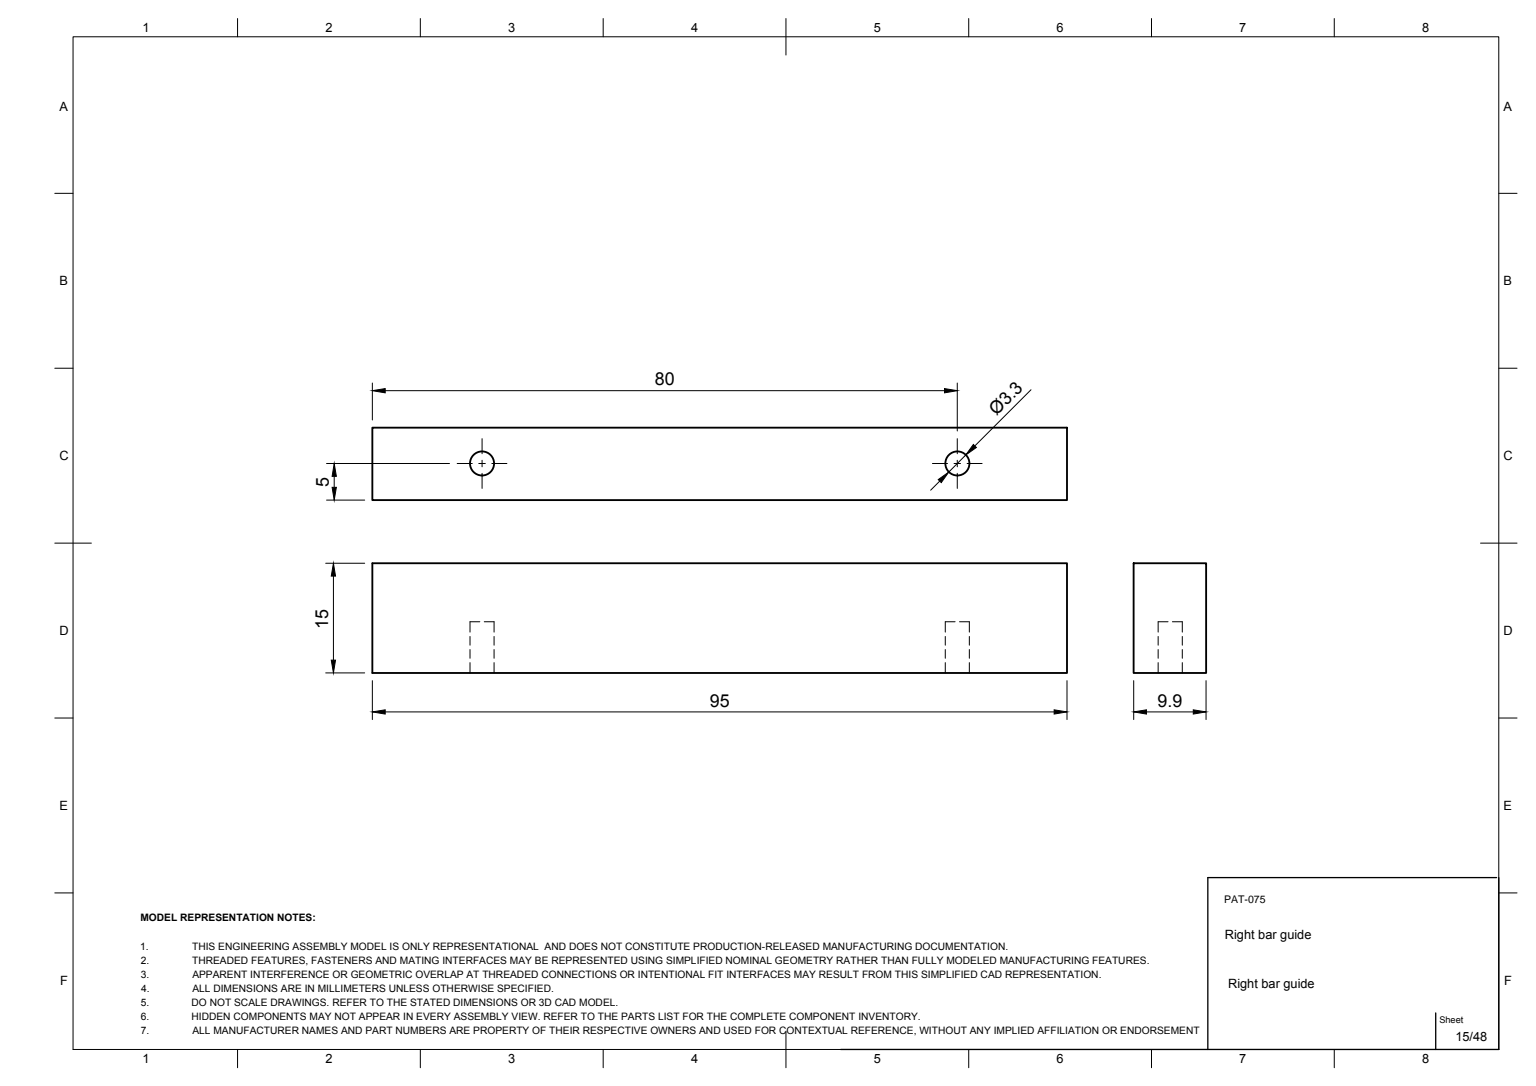
ISO-10303-21;
HEADER;
/* Generated by software containing ST-Developer
 * from STEP Tools, Inc. (www.steptools.com) 
 */

FILE_DESCRIPTION(
/* description */ ('Over-Centre Plunger Toggle Clamp on Slotted Fixture Frame'),
/* implementation_level */ '2;1');

FILE_NAME(
/* name */ 
'Right bar guide.step',
/* time_stamp */ '2026-10-28T03:23:24-07:00',
/* author */ (''),
/* organization */ (''),
/* preprocessor_version */ 'ST-DEVELOPER v20.2',
/* originating_system */ 'Autodesk Translation Framework v15.17.0.0',
/* authorisation */ '');

FILE_SCHEMA (('AUTOMOTIVE_DESIGN { 1 0 10303 214 3 1 1 }'));
ENDSEC;

DATA;
#10=MECHANICAL_DESIGN_GEOMETRIC_PRESENTATION_REPRESENTATION('',(#523),#15212);
#439=SHAPE_REPRESENTATION_RELATIONSHIP('SRR','None',#15413,#481);
#481=ADVANCED_BREP_SHAPE_REPRESENTATION('',(#574),#15175);
#523=STYLED_ITEM('',(#15733),#574);
#574=MANIFOLD_SOLID_BREP('Body1',#8255);
#710=FACE_BOUND('',#1814,.T.);
#711=FACE_BOUND('',#1815,.T.);
#854=PLANE('',#9033);
#855=PLANE('',#9037);
#856=PLANE('',#9038);
#857=PLANE('',#9039);
#858=PLANE('',#9040);
#859=PLANE('',#9041);
#860=PLANE('',#9042);
#861=PLANE('',#9043);
#1219=FACE_OUTER_BOUND('',#1804,.T.);
#1220=FACE_OUTER_BOUND('',#1805,.T.);
#1221=FACE_OUTER_BOUND('',#1806,.T.);
#1222=FACE_OUTER_BOUND('',#1807,.T.);
#1223=FACE_OUTER_BOUND('',#1808,.T.);
#1224=FACE_OUTER_BOUND('',#1809,.T.);
#1225=FACE_OUTER_BOUND('',#1810,.T.);
#1226=FACE_OUTER_BOUND('',#1811,.T.);
#1227=FACE_OUTER_BOUND('',#1812,.T.);
#1228=FACE_OUTER_BOUND('',#1813,.T.);
#1804=EDGE_LOOP('',(#6151,#6152,#6153,#6154));
#1805=EDGE_LOOP('',(#6155));
#1806=EDGE_LOOP('',(#6156,#6157,#6158,#6159));
#1807=EDGE_LOOP('',(#6160));
#1808=EDGE_LOOP('',(#6161,#6162,#6163,#6164));
#1809=EDGE_LOOP('',(#6165,#6166,#6167,#6168));
#1810=EDGE_LOOP('',(#6169,#6170,#6171,#6172));
#1811=EDGE_LOOP('',(#6173,#6174,#6175,#6176));
#1812=EDGE_LOOP('',(#6177,#6178,#6179,#6180));
#1813=EDGE_LOOP('',(#6181,#6182,#6183,#6184));
#1814=EDGE_LOOP('',(#6185));
#1815=EDGE_LOOP('',(#6186));
#2400=LINE('',#13000,#3030);
#2401=LINE('',#13007,#3031);
#2402=LINE('',#13013,#3032);
#2403=LINE('',#13015,#3033);
#2404=LINE('',#13017,#3034);
#2405=LINE('',#13018,#3035);
#2406=LINE('',#13021,#3036);
#2407=LINE('',#13023,#3037);
#2408=LINE('',#13024,#3038);
#2409=LINE('',#13027,#3039);
#2410=LINE('',#13029,#3040);
#2411=LINE('',#13030,#3041);
#2412=LINE('',#13032,#3042);
#2413=LINE('',#13033,#3043);
#3030=VECTOR('',#10461,0.165);
#3031=VECTOR('',#10470,0.165);
#3032=VECTOR('',#10477,1.);
#3033=VECTOR('',#10478,1.);
#3034=VECTOR('',#10479,1.);
#3035=VECTOR('',#10480,1.);
#3036=VECTOR('',#10483,1.);
#3037=VECTOR('',#10484,1.);
#3038=VECTOR('',#10485,1.);
#3039=VECTOR('',#10488,1.);
#3040=VECTOR('',#10489,1.);
#3041=VECTOR('',#10490,1.);
#3042=VECTOR('',#10493,1.);
#3043=VECTOR('',#10494,1.);
#3613=CIRCLE('',#9031,0.165);
#3614=CIRCLE('',#9032,0.165);
#3615=CIRCLE('',#9035,0.165);
#3616=CIRCLE('',#9036,0.165);
#4053=VERTEX_POINT('',#12997);
#4054=VERTEX_POINT('',#12999);
#4055=VERTEX_POINT('',#13004);
#4056=VERTEX_POINT('',#13006);
#4057=VERTEX_POINT('',#13011);
#4058=VERTEX_POINT('',#13012);
#4059=VERTEX_POINT('',#13014);
#4060=VERTEX_POINT('',#13016);
#4061=VERTEX_POINT('',#13020);
#4062=VERTEX_POINT('',#13022);
#4063=VERTEX_POINT('',#13026);
#4064=VERTEX_POINT('',#13028);
#4836=EDGE_CURVE('',#4053,#4053,#3613,.T.);
#4837=EDGE_CURVE('',#4053,#4054,#2400,.T.);
#4838=EDGE_CURVE('',#4054,#4054,#3614,.T.);
#4839=EDGE_CURVE('',#4055,#4055,#3615,.T.);
#4840=EDGE_CURVE('',#4055,#4056,#2401,.T.);
#4841=EDGE_CURVE('',#4056,#4056,#3616,.T.);
#4842=EDGE_CURVE('',#4057,#4058,#2402,.T.);
#4843=EDGE_CURVE('',#4058,#4059,#2403,.T.);
#4844=EDGE_CURVE('',#4060,#4059,#2404,.T.);
#4845=EDGE_CURVE('',#4057,#4060,#2405,.T.);
#4846=EDGE_CURVE('',#4061,#4057,#2406,.T.);
#4847=EDGE_CURVE('',#4062,#4060,#2407,.T.);
#4848=EDGE_CURVE('',#4061,#4062,#2408,.T.);
#4849=EDGE_CURVE('',#4063,#4061,#2409,.T.);
#4850=EDGE_CURVE('',#4064,#4062,#2410,.T.);
#4851=EDGE_CURVE('',#4063,#4064,#2411,.T.);
#4852=EDGE_CURVE('',#4058,#4063,#2412,.T.);
#4853=EDGE_CURVE('',#4059,#4064,#2413,.T.);
#6151=ORIENTED_EDGE('',*,*,#4836,.F.);
#6152=ORIENTED_EDGE('',*,*,#4837,.T.);
#6153=ORIENTED_EDGE('',*,*,#4838,.T.);
#6154=ORIENTED_EDGE('',*,*,#4837,.F.);
#6155=ORIENTED_EDGE('',*,*,#4838,.F.);
#6156=ORIENTED_EDGE('',*,*,#4839,.F.);
#6157=ORIENTED_EDGE('',*,*,#4840,.T.);
#6158=ORIENTED_EDGE('',*,*,#4841,.T.);
#6159=ORIENTED_EDGE('',*,*,#4840,.F.);
#6160=ORIENTED_EDGE('',*,*,#4841,.F.);
#6161=ORIENTED_EDGE('',*,*,#4842,.T.);
#6162=ORIENTED_EDGE('',*,*,#4843,.T.);
#6163=ORIENTED_EDGE('',*,*,#4844,.F.);
#6164=ORIENTED_EDGE('',*,*,#4845,.F.);
#6165=ORIENTED_EDGE('',*,*,#4846,.T.);
#6166=ORIENTED_EDGE('',*,*,#4845,.T.);
#6167=ORIENTED_EDGE('',*,*,#4847,.F.);
#6168=ORIENTED_EDGE('',*,*,#4848,.F.);
#6169=ORIENTED_EDGE('',*,*,#4849,.T.);
#6170=ORIENTED_EDGE('',*,*,#4848,.T.);
#6171=ORIENTED_EDGE('',*,*,#4850,.F.);
#6172=ORIENTED_EDGE('',*,*,#4851,.F.);
#6173=ORIENTED_EDGE('',*,*,#4852,.T.);
#6174=ORIENTED_EDGE('',*,*,#4851,.T.);
#6175=ORIENTED_EDGE('',*,*,#4853,.F.);
#6176=ORIENTED_EDGE('',*,*,#4843,.F.);
#6177=ORIENTED_EDGE('',*,*,#4853,.T.);
#6178=ORIENTED_EDGE('',*,*,#4850,.T.);
#6179=ORIENTED_EDGE('',*,*,#4847,.T.);
#6180=ORIENTED_EDGE('',*,*,#4844,.T.);
#6181=ORIENTED_EDGE('',*,*,#4852,.F.);
#6182=ORIENTED_EDGE('',*,*,#4842,.F.);
#6183=ORIENTED_EDGE('',*,*,#4846,.F.);
#6184=ORIENTED_EDGE('',*,*,#4849,.F.);
#6185=ORIENTED_EDGE('',*,*,#4836,.T.);
#6186=ORIENTED_EDGE('',*,*,#4839,.T.);
#7678=CYLINDRICAL_SURFACE('',#9030,0.165);
#7679=CYLINDRICAL_SURFACE('',#9034,0.165);
#7891=ADVANCED_FACE('',(#1219),#7678,.F.);
#7892=ADVANCED_FACE('',(#1220),#854,.F.);
#7893=ADVANCED_FACE('',(#1221),#7679,.F.);
#7894=ADVANCED_FACE('',(#1222),#855,.F.);
#7895=ADVANCED_FACE('',(#1223),#856,.T.);
#7896=ADVANCED_FACE('',(#1224),#857,.T.);
#7897=ADVANCED_FACE('',(#1225),#858,.T.);
#7898=ADVANCED_FACE('',(#1226),#859,.T.);
#7899=ADVANCED_FACE('',(#1227),#860,.T.);
#7900=ADVANCED_FACE('',(#1228,#710,#711),#861,.F.);
#8255=CLOSED_SHELL('',(#7891,#7892,#7893,#7894,#7895,#7896,#7897,#7898,
#7899,#7900));
#9029=AXIS2_PLACEMENT_3D('',#12995,#10455,#10456);
#9030=AXIS2_PLACEMENT_3D('',#12996,#10457,#10458);
#9031=AXIS2_PLACEMENT_3D('',#12998,#10459,#10460);
#9032=AXIS2_PLACEMENT_3D('',#13001,#10462,#10463);
#9033=AXIS2_PLACEMENT_3D('',#13002,#10464,#10465);
#9034=AXIS2_PLACEMENT_3D('',#13003,#10466,#10467);
#9035=AXIS2_PLACEMENT_3D('',#13005,#10468,#10469);
#9036=AXIS2_PLACEMENT_3D('',#13008,#10471,#10472);
#9037=AXIS2_PLACEMENT_3D('',#13009,#10473,#10474);
#9038=AXIS2_PLACEMENT_3D('',#13010,#10475,#10476);
#9039=AXIS2_PLACEMENT_3D('',#13019,#10481,#10482);
#9040=AXIS2_PLACEMENT_3D('',#13025,#10486,#10487);
#9041=AXIS2_PLACEMENT_3D('',#13031,#10491,#10492);
#9042=AXIS2_PLACEMENT_3D('',#13034,#10495,#10496);
#9043=AXIS2_PLACEMENT_3D('',#13035,#10497,#10498);
#10455=DIRECTION('axis',(0.,0.,1.));
#10456=DIRECTION('refdir',(1.,0.,0.));
#10457=DIRECTION('center_axis',(0.,0.,1.));
#10458=DIRECTION('ref_axis',(1.,0.,0.));
#10459=DIRECTION('center_axis',(0.,0.,1.));
#10460=DIRECTION('ref_axis',(1.,0.,0.));
#10461=DIRECTION('',(0.,0.,1.));
#10462=DIRECTION('center_axis',(0.,0.,1.));
#10463=DIRECTION('ref_axis',(1.,0.,0.));
#10464=DIRECTION('center_axis',(0.,0.,1.));
#10465=DIRECTION('ref_axis',(1.,0.,0.));
#10466=DIRECTION('center_axis',(0.,0.,1.));
#10467=DIRECTION('ref_axis',(1.,0.,0.));
#10468=DIRECTION('center_axis',(0.,0.,1.));
#10469=DIRECTION('ref_axis',(1.,0.,0.));
#10470=DIRECTION('',(0.,0.,1.));
#10471=DIRECTION('center_axis',(0.,0.,1.));
#10472=DIRECTION('ref_axis',(1.,0.,0.));
#10473=DIRECTION('center_axis',(0.,0.,1.));
#10474=DIRECTION('ref_axis',(1.,0.,0.));
#10475=DIRECTION('center_axis',(0.,1.,0.));
#10476=DIRECTION('ref_axis',(-1.,0.,0.));
#10477=DIRECTION('',(-1.,0.,0.));
#10478=DIRECTION('',(0.,0.,1.));
#10479=DIRECTION('',(-1.,0.,0.));
#10480=DIRECTION('',(0.,0.,1.));
#10481=DIRECTION('center_axis',(1.,0.,0.));
#10482=DIRECTION('ref_axis',(0.,1.,0.));
#10483=DIRECTION('',(0.,1.,0.));
#10484=DIRECTION('',(0.,1.,0.));
#10485=DIRECTION('',(0.,0.,1.));
#10486=DIRECTION('center_axis',(0.,-1.,0.));
#10487=DIRECTION('ref_axis',(1.,0.,0.));
#10488=DIRECTION('',(1.,0.,0.));
#10489=DIRECTION('',(1.,0.,0.));
#10490=DIRECTION('',(0.,0.,1.));
#10491=DIRECTION('center_axis',(-1.,0.,0.));
#10492=DIRECTION('ref_axis',(0.,-1.,0.));
#10493=DIRECTION('',(0.,-1.,0.));
#10494=DIRECTION('',(0.,-1.,0.));
#10495=DIRECTION('center_axis',(0.,0.,1.));
#10496=DIRECTION('ref_axis',(1.,0.,0.));
#10497=DIRECTION('center_axis',(0.,0.,1.));
#10498=DIRECTION('ref_axis',(1.,0.,0.));
#12995=CARTESIAN_POINT('',(0.,0.,0.));
#12996=CARTESIAN_POINT('Origin',(1.5,-4.5,0.9));
#12997=CARTESIAN_POINT('',(1.335,-4.5,1.));
#12998=CARTESIAN_POINT('Origin',(1.5,-4.5,1.));
#12999=CARTESIAN_POINT('',(1.335,-4.5,1.7));
#13000=CARTESIAN_POINT('',(1.335,-4.5,0.9));
#13001=CARTESIAN_POINT('Origin',(1.5,-4.5,1.7));
#13002=CARTESIAN_POINT('Origin',(1.5,-4.5,1.7));
#13003=CARTESIAN_POINT('Origin',(1.5,2.,0.9));
#13004=CARTESIAN_POINT('',(1.335,2.,1.));
#13005=CARTESIAN_POINT('Origin',(1.5,2.,1.));
#13006=CARTESIAN_POINT('',(1.335,2.,1.7));
#13007=CARTESIAN_POINT('',(1.335,2.,0.9));
#13008=CARTESIAN_POINT('Origin',(1.5,2.,1.7));
#13009=CARTESIAN_POINT('Origin',(1.5,2.,1.7));
#13010=CARTESIAN_POINT('Origin',(2.,3.5,1.));
#13011=CARTESIAN_POINT('',(2.,3.5,1.));
#13012=CARTESIAN_POINT('',(1.01,3.5,1.));
#13013=CARTESIAN_POINT('',(2.,3.5,1.));
#13014=CARTESIAN_POINT('',(1.01,3.5,2.5));
#13015=CARTESIAN_POINT('',(1.01,3.5,1.));
#13016=CARTESIAN_POINT('',(2.,3.5,2.5));
#13017=CARTESIAN_POINT('',(2.,3.5,2.5));
#13018=CARTESIAN_POINT('',(2.,3.5,1.));
#13019=CARTESIAN_POINT('Origin',(2.,-6.,1.));
#13020=CARTESIAN_POINT('',(2.,-6.,1.));
#13021=CARTESIAN_POINT('',(2.,-6.,1.));
#13022=CARTESIAN_POINT('',(2.,-6.,2.5));
#13023=CARTESIAN_POINT('',(2.,-6.,2.5));
#13024=CARTESIAN_POINT('',(2.,-6.,1.));
#13025=CARTESIAN_POINT('Origin',(1.01,-6.,1.));
#13026=CARTESIAN_POINT('',(1.01,-6.,1.));
#13027=CARTESIAN_POINT('',(1.01,-6.,1.));
#13028=CARTESIAN_POINT('',(1.01,-6.,2.5));
#13029=CARTESIAN_POINT('',(1.01,-6.,2.5));
#13030=CARTESIAN_POINT('',(1.01,-6.,1.));
#13031=CARTESIAN_POINT('Origin',(1.01,3.5,1.));
#13032=CARTESIAN_POINT('',(1.01,3.5,1.));
#13033=CARTESIAN_POINT('',(1.01,3.5,2.5));
#13034=CARTESIAN_POINT('Origin',(1.505,-1.25,2.5));
#13035=CARTESIAN_POINT('Origin',(1.505,-1.25,1.));
#15125=UNCERTAINTY_MEASURE_WITH_UNIT(LENGTH_MEASURE(0.001),#15213,
'DISTANCE_ACCURACY_VALUE',
'Maximum model space distance between geometric entities at asserted c
onnectivities');
#15162=UNCERTAINTY_MEASURE_WITH_UNIT(LENGTH_MEASURE(0.001),#15213,
'DISTANCE_ACCURACY_VALUE',
'Maximum model space distance between geometric entities at asserted c
onnectivities');
#15175=(
GEOMETRIC_REPRESENTATION_CONTEXT(3)
GLOBAL_UNCERTAINTY_ASSIGNED_CONTEXT((#15125))
GLOBAL_UNIT_ASSIGNED_CONTEXT((#15213,#15215,#15216))
REPRESENTATION_CONTEXT('','3D')
);
#15212=(
GEOMETRIC_REPRESENTATION_CONTEXT(3)
GLOBAL_UNCERTAINTY_ASSIGNED_CONTEXT((#15162))
GLOBAL_UNIT_ASSIGNED_CONTEXT((#15213,#15215,#15216))
REPRESENTATION_CONTEXT('','3D')
);
#15213=(
LENGTH_UNIT()
NAMED_UNIT(*)
SI_UNIT(.CENTI.,.METRE.)
);
#15215=(
NAMED_UNIT(*)
PLANE_ANGLE_UNIT()
SI_UNIT($,.RADIAN.)
);
#15216=(
NAMED_UNIT(*)
SI_UNIT($,.STERADIAN.)
SOLID_ANGLE_UNIT()
);
#15229=SHAPE_DEFINITION_REPRESENTATION(#15278,#15413);
#15278=PRODUCT_DEFINITION_SHAPE('',$,#15463);
#15413=SHAPE_REPRESENTATION('',(#9029),#15175);
#15450=PRODUCT_DEFINITION_CONTEXT('part definition',#15599,'design');
#15463=PRODUCT_DEFINITION('Right bar guide','Right bar guide',#15512,#15450);
#15512=PRODUCT_DEFINITION_FORMATION('',$,#15613);
#15599=APPLICATION_CONTEXT(
'Core Data for Automotive Mechanical Design Process');
#15600=PRODUCT_CONTEXT('part definition',#15599,'mechanical');
#15613=PRODUCT('Right bar guide','Right bar guide','Right bar guide',(#15600));
#15727=COLOUR_RGB('Off White',0.89,0.88,0.83);
#15728=FILL_AREA_STYLE_COLOUR('',#15727);
#15729=FILL_AREA_STYLE('',(#15728));
#15730=SURFACE_STYLE_FILL_AREA(#15729);
#15731=SURFACE_SIDE_STYLE('',(#15730));
#15732=SURFACE_STYLE_USAGE(.BOTH.,#15731);
#15733=PRESENTATION_STYLE_ASSIGNMENT((#15732));
ENDSEC;
END-ISO-10303-21;
